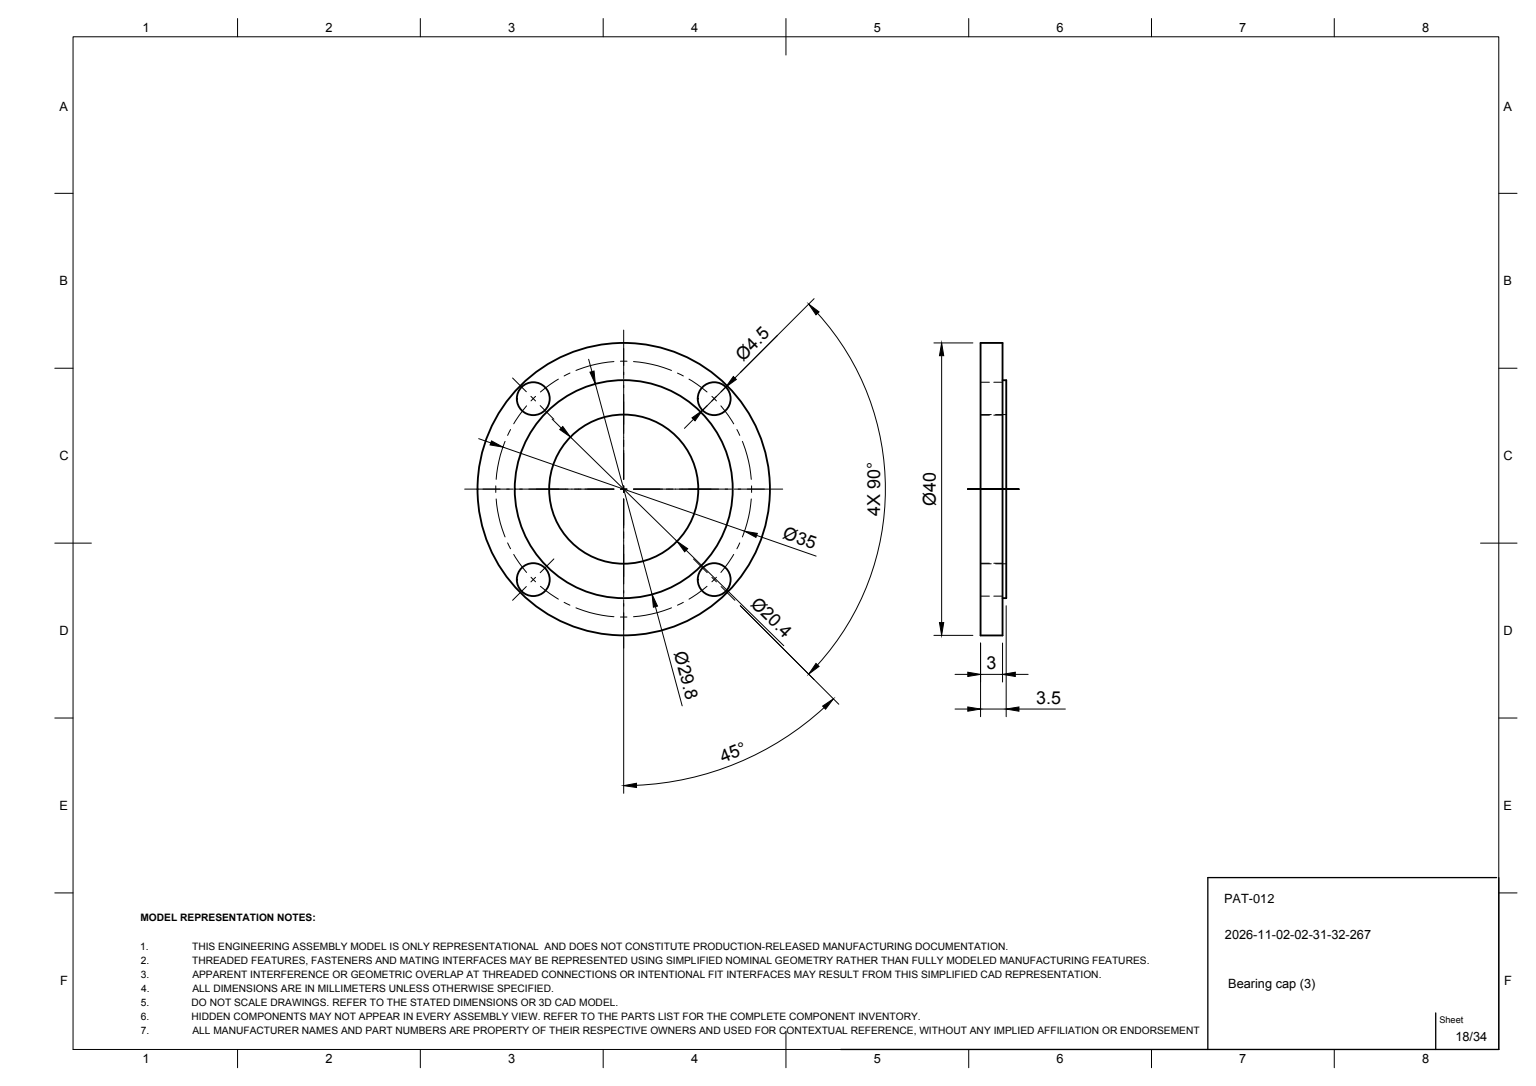
ISO-10303-21;
HEADER;
/* Generated by software containing ST-Developer
 * from STEP Tools, Inc. (www.steptools.com) 
 */

FILE_DESCRIPTION(
/* description */ ('Belt tensioner idler arm'),
/* implementation_level */ '2;1');

FILE_NAME(
/* name */ 'Bearing cap (3).step',
/* time_stamp */ '2026-10-28T03:22:15-07:00',
/* author */ (''),
/* organization */ (''),
/* preprocessor_version */ 'ST-DEVELOPER v20.2',
/* originating_system */ 'Autodesk Translation Framework v15.17.0.0',
/* authorisation */ '');

FILE_SCHEMA (('AUTOMOTIVE_DESIGN { 1 0 10303 214 3 1 1 }'));
ENDSEC;

DATA;
#10=MECHANICAL_DESIGN_GEOMETRIC_PRESENTATION_REPRESENTATION('',(#463),#12779);
#395=SHAPE_REPRESENTATION_RELATIONSHIP('SRR','None',#12942,#429);
#429=ADVANCED_BREP_SHAPE_REPRESENTATION('',(#503),#12759);
#463=STYLED_ITEM('',(#13184),#503);
#503=MANIFOLD_SOLID_BREP('Body1',#6199);
#615=FACE_BOUND('',#1463,.T.);
#616=FACE_BOUND('',#1467,.T.);
#617=FACE_BOUND('',#1468,.T.);
#618=FACE_BOUND('',#1469,.T.);
#619=FACE_BOUND('',#1470,.T.);
#620=FACE_BOUND('',#1471,.T.);
#621=FACE_BOUND('',#1473,.T.);
#622=FACE_BOUND('',#1474,.T.);
#623=FACE_BOUND('',#1475,.T.);
#624=FACE_BOUND('',#1476,.T.);
#625=FACE_BOUND('',#1477,.T.);
#753=PLANE('',#6941);
#754=PLANE('',#6948);
#755=PLANE('',#6949);
#1002=FACE_OUTER_BOUND('',#1457,.T.);
#1003=FACE_OUTER_BOUND('',#1458,.T.);
#1004=FACE_OUTER_BOUND('',#1459,.T.);
#1005=FACE_OUTER_BOUND('',#1460,.T.);
#1006=FACE_OUTER_BOUND('',#1461,.T.);
#1007=FACE_OUTER_BOUND('',#1462,.T.);
#1008=FACE_OUTER_BOUND('',#1464,.T.);
#1009=FACE_OUTER_BOUND('',#1465,.T.);
#1010=FACE_OUTER_BOUND('',#1466,.T.);
#1011=FACE_OUTER_BOUND('',#1472,.T.);
#1457=EDGE_LOOP('',(#4764,#4765,#4766,#4767));
#1458=EDGE_LOOP('',(#4768,#4769,#4770,#4771));
#1459=EDGE_LOOP('',(#4772,#4773,#4774,#4775));
#1460=EDGE_LOOP('',(#4776,#4777,#4778,#4779));
#1461=EDGE_LOOP('',(#4780,#4781,#4782,#4783));
#1462=EDGE_LOOP('',(#4784));
#1463=EDGE_LOOP('',(#4785));
#1464=EDGE_LOOP('',(#4786,#4787,#4788,#4789));
#1465=EDGE_LOOP('',(#4790,#4791,#4792,#4793));
#1466=EDGE_LOOP('',(#4794));
#1467=EDGE_LOOP('',(#4795));
#1468=EDGE_LOOP('',(#4796));
#1469=EDGE_LOOP('',(#4797));
#1470=EDGE_LOOP('',(#4798));
#1471=EDGE_LOOP('',(#4799));
#1472=EDGE_LOOP('',(#4800));
#1473=EDGE_LOOP('',(#4801));
#1474=EDGE_LOOP('',(#4802));
#1475=EDGE_LOOP('',(#4803));
#1476=EDGE_LOOP('',(#4804));
#1477=EDGE_LOOP('',(#4805));
#1882=LINE('',#10918,#2231);
#1883=LINE('',#10924,#2232);
#1884=LINE('',#10930,#2233);
#1885=LINE('',#10936,#2234);
#1886=LINE('',#10942,#2235);
#1887=LINE('',#10950,#2236);
#1888=LINE('',#10955,#2237);
#2231=VECTOR('',#8260,0.225);
#2232=VECTOR('',#8267,0.225);
#2233=VECTOR('',#8274,0.225);
#2234=VECTOR('',#8281,0.225);
#2235=VECTOR('',#8288,1.49);
#2236=VECTOR('',#8299,1.02);
#2237=VECTOR('',#8304,2.);
#2544=CIRCLE('',#6927,0.225);
#2545=CIRCLE('',#6928,0.225);
#2546=CIRCLE('',#6930,0.225);
#2547=CIRCLE('',#6931,0.225);
#2548=CIRCLE('',#6933,0.225);
#2549=CIRCLE('',#6934,0.225);
#2550=CIRCLE('',#6936,0.225);
#2551=CIRCLE('',#6937,0.225);
#2552=CIRCLE('',#6939,1.49);
#2553=CIRCLE('',#6940,1.49);
#2554=CIRCLE('',#6942,1.02);
#2555=CIRCLE('',#6944,1.02);
#2556=CIRCLE('',#6946,2.);
#2557=CIRCLE('',#6947,2.);
#2989=VERTEX_POINT('',#10915);
#2990=VERTEX_POINT('',#10917);
#2991=VERTEX_POINT('',#10921);
#2992=VERTEX_POINT('',#10923);
#2993=VERTEX_POINT('',#10927);
#2994=VERTEX_POINT('',#10929);
#2995=VERTEX_POINT('',#10933);
#2996=VERTEX_POINT('',#10935);
#2997=VERTEX_POINT('',#10939);
#2998=VERTEX_POINT('',#10941);
#2999=VERTEX_POINT('',#10945);
#3000=VERTEX_POINT('',#10948);
#3001=VERTEX_POINT('',#10952);
#3002=VERTEX_POINT('',#10954);
#3637=EDGE_CURVE('',#2989,#2989,#2544,.T.);
#3638=EDGE_CURVE('',#2989,#2990,#1882,.T.);
#3639=EDGE_CURVE('',#2990,#2990,#2545,.T.);
#3640=EDGE_CURVE('',#2991,#2991,#2546,.T.);
#3641=EDGE_CURVE('',#2991,#2992,#1883,.T.);
#3642=EDGE_CURVE('',#2992,#2992,#2547,.T.);
#3643=EDGE_CURVE('',#2993,#2993,#2548,.T.);
#3644=EDGE_CURVE('',#2993,#2994,#1884,.T.);
#3645=EDGE_CURVE('',#2994,#2994,#2549,.T.);
#3646=EDGE_CURVE('',#2995,#2995,#2550,.T.);
#3647=EDGE_CURVE('',#2995,#2996,#1885,.T.);
#3648=EDGE_CURVE('',#2996,#2996,#2551,.T.);
#3649=EDGE_CURVE('',#2997,#2997,#2552,.T.);
#3650=EDGE_CURVE('',#2997,#2998,#1886,.T.);
#3651=EDGE_CURVE('',#2998,#2998,#2553,.T.);
#3652=EDGE_CURVE('',#2999,#2999,#2554,.T.);
#3653=EDGE_CURVE('',#3000,#3000,#2555,.T.);
#3654=EDGE_CURVE('',#3000,#2999,#1887,.T.);
#3655=EDGE_CURVE('',#3001,#3001,#2556,.T.);
#3656=EDGE_CURVE('',#3001,#3002,#1888,.T.);
#3657=EDGE_CURVE('',#3002,#3002,#2557,.T.);
#4764=ORIENTED_EDGE('',*,*,#3637,.F.);
#4765=ORIENTED_EDGE('',*,*,#3638,.T.);
#4766=ORIENTED_EDGE('',*,*,#3639,.F.);
#4767=ORIENTED_EDGE('',*,*,#3638,.F.);
#4768=ORIENTED_EDGE('',*,*,#3640,.F.);
#4769=ORIENTED_EDGE('',*,*,#3641,.T.);
#4770=ORIENTED_EDGE('',*,*,#3642,.F.);
#4771=ORIENTED_EDGE('',*,*,#3641,.F.);
#4772=ORIENTED_EDGE('',*,*,#3643,.F.);
#4773=ORIENTED_EDGE('',*,*,#3644,.T.);
#4774=ORIENTED_EDGE('',*,*,#3645,.F.);
#4775=ORIENTED_EDGE('',*,*,#3644,.F.);
#4776=ORIENTED_EDGE('',*,*,#3646,.F.);
#4777=ORIENTED_EDGE('',*,*,#3647,.T.);
#4778=ORIENTED_EDGE('',*,*,#3648,.F.);
#4779=ORIENTED_EDGE('',*,*,#3647,.F.);
#4780=ORIENTED_EDGE('',*,*,#3649,.F.);
#4781=ORIENTED_EDGE('',*,*,#3650,.T.);
#4782=ORIENTED_EDGE('',*,*,#3651,.T.);
#4783=ORIENTED_EDGE('',*,*,#3650,.F.);
#4784=ORIENTED_EDGE('',*,*,#3651,.F.);
#4785=ORIENTED_EDGE('',*,*,#3652,.F.);
#4786=ORIENTED_EDGE('',*,*,#3653,.F.);
#4787=ORIENTED_EDGE('',*,*,#3654,.T.);
#4788=ORIENTED_EDGE('',*,*,#3652,.T.);
#4789=ORIENTED_EDGE('',*,*,#3654,.F.);
#4790=ORIENTED_EDGE('',*,*,#3655,.F.);
#4791=ORIENTED_EDGE('',*,*,#3656,.T.);
#4792=ORIENTED_EDGE('',*,*,#3657,.T.);
#4793=ORIENTED_EDGE('',*,*,#3656,.F.);
#4794=ORIENTED_EDGE('',*,*,#3655,.T.);
#4795=ORIENTED_EDGE('',*,*,#3653,.T.);
#4796=ORIENTED_EDGE('',*,*,#3648,.T.);
#4797=ORIENTED_EDGE('',*,*,#3645,.T.);
#4798=ORIENTED_EDGE('',*,*,#3642,.T.);
#4799=ORIENTED_EDGE('',*,*,#3639,.T.);
#4800=ORIENTED_EDGE('',*,*,#3657,.F.);
#4801=ORIENTED_EDGE('',*,*,#3649,.T.);
#4802=ORIENTED_EDGE('',*,*,#3646,.T.);
#4803=ORIENTED_EDGE('',*,*,#3643,.T.);
#4804=ORIENTED_EDGE('',*,*,#3640,.T.);
#4805=ORIENTED_EDGE('',*,*,#3637,.T.);
#5725=CYLINDRICAL_SURFACE('',#6926,0.225);
#5726=CYLINDRICAL_SURFACE('',#6929,0.225);
#5727=CYLINDRICAL_SURFACE('',#6932,0.225);
#5728=CYLINDRICAL_SURFACE('',#6935,0.225);
#5729=CYLINDRICAL_SURFACE('',#6938,1.49);
#5730=CYLINDRICAL_SURFACE('',#6943,1.02);
#5731=CYLINDRICAL_SURFACE('',#6945,2.);
#5979=ADVANCED_FACE('',(#1002),#5725,.F.);
#5980=ADVANCED_FACE('',(#1003),#5726,.F.);
#5981=ADVANCED_FACE('',(#1004),#5727,.F.);
#5982=ADVANCED_FACE('',(#1005),#5728,.F.);
#5983=ADVANCED_FACE('',(#1006),#5729,.T.);
#5984=ADVANCED_FACE('',(#1007,#615),#753,.F.);
#5985=ADVANCED_FACE('',(#1008),#5730,.F.);
#5986=ADVANCED_FACE('',(#1009),#5731,.T.);
#5987=ADVANCED_FACE('',(#1010,#616,#617,#618,#619,#620),#754,.T.);
#5988=ADVANCED_FACE('',(#1011,#621,#622,#623,#624,#625),#755,.F.);
#6199=CLOSED_SHELL('',(#5979,#5980,#5981,#5982,#5983,#5984,#5985,#5986,
#5987,#5988));
#6925=AXIS2_PLACEMENT_3D('',#10913,#8254,#8255);
#6926=AXIS2_PLACEMENT_3D('',#10914,#8256,#8257);
#6927=AXIS2_PLACEMENT_3D('',#10916,#8258,#8259);
#6928=AXIS2_PLACEMENT_3D('',#10919,#8261,#8262);
#6929=AXIS2_PLACEMENT_3D('',#10920,#8263,#8264);
#6930=AXIS2_PLACEMENT_3D('',#10922,#8265,#8266);
#6931=AXIS2_PLACEMENT_3D('',#10925,#8268,#8269);
#6932=AXIS2_PLACEMENT_3D('',#10926,#8270,#8271);
#6933=AXIS2_PLACEMENT_3D('',#10928,#8272,#8273);
#6934=AXIS2_PLACEMENT_3D('',#10931,#8275,#8276);
#6935=AXIS2_PLACEMENT_3D('',#10932,#8277,#8278);
#6936=AXIS2_PLACEMENT_3D('',#10934,#8279,#8280);
#6937=AXIS2_PLACEMENT_3D('',#10937,#8282,#8283);
#6938=AXIS2_PLACEMENT_3D('',#10938,#8284,#8285);
#6939=AXIS2_PLACEMENT_3D('',#10940,#8286,#8287);
#6940=AXIS2_PLACEMENT_3D('',#10943,#8289,#8290);
#6941=AXIS2_PLACEMENT_3D('',#10944,#8291,#8292);
#6942=AXIS2_PLACEMENT_3D('',#10946,#8293,#8294);
#6943=AXIS2_PLACEMENT_3D('',#10947,#8295,#8296);
#6944=AXIS2_PLACEMENT_3D('',#10949,#8297,#8298);
#6945=AXIS2_PLACEMENT_3D('',#10951,#8300,#8301);
#6946=AXIS2_PLACEMENT_3D('',#10953,#8302,#8303);
#6947=AXIS2_PLACEMENT_3D('',#10956,#8305,#8306);
#6948=AXIS2_PLACEMENT_3D('',#10957,#8307,#8308);
#6949=AXIS2_PLACEMENT_3D('',#10958,#8309,#8310);
#8254=DIRECTION('axis',(0.,0.,1.));
#8255=DIRECTION('refdir',(1.,0.,0.));
#8256=DIRECTION('center_axis',(0.,0.,1.));
#8257=DIRECTION('ref_axis',(1.,0.,0.));
#8258=DIRECTION('center_axis',(0.,0.,1.));
#8259=DIRECTION('ref_axis',(1.,0.,0.));
#8260=DIRECTION('',(0.,0.,1.));
#8261=DIRECTION('center_axis',(0.,0.,-1.));
#8262=DIRECTION('ref_axis',(1.,0.,0.));
#8263=DIRECTION('center_axis',(0.,0.,1.));
#8264=DIRECTION('ref_axis',(1.,0.,0.));
#8265=DIRECTION('center_axis',(0.,0.,1.));
#8266=DIRECTION('ref_axis',(1.,0.,0.));
#8267=DIRECTION('',(0.,0.,1.));
#8268=DIRECTION('center_axis',(0.,0.,-1.));
#8269=DIRECTION('ref_axis',(1.,0.,0.));
#8270=DIRECTION('center_axis',(0.,0.,1.));
#8271=DIRECTION('ref_axis',(1.,0.,0.));
#8272=DIRECTION('center_axis',(0.,0.,1.));
#8273=DIRECTION('ref_axis',(1.,0.,0.));
#8274=DIRECTION('',(0.,0.,1.));
#8275=DIRECTION('center_axis',(0.,0.,-1.));
#8276=DIRECTION('ref_axis',(1.,0.,0.));
#8277=DIRECTION('center_axis',(0.,0.,1.));
#8278=DIRECTION('ref_axis',(1.,0.,0.));
#8279=DIRECTION('center_axis',(0.,0.,1.));
#8280=DIRECTION('ref_axis',(1.,0.,0.));
#8281=DIRECTION('',(0.,0.,1.));
#8282=DIRECTION('center_axis',(0.,0.,-1.));
#8283=DIRECTION('ref_axis',(1.,0.,0.));
#8284=DIRECTION('center_axis',(0.,0.,1.));
#8285=DIRECTION('ref_axis',(1.,0.,0.));
#8286=DIRECTION('center_axis',(0.,0.,1.));
#8287=DIRECTION('ref_axis',(1.,0.,0.));
#8288=DIRECTION('',(0.,0.,-1.));
#8289=DIRECTION('center_axis',(0.,0.,1.));
#8290=DIRECTION('ref_axis',(1.,0.,0.));
#8291=DIRECTION('center_axis',(0.,0.,1.));
#8292=DIRECTION('ref_axis',(1.,0.,0.));
#8293=DIRECTION('center_axis',(0.,0.,-1.));
#8294=DIRECTION('ref_axis',(1.,0.,0.));
#8295=DIRECTION('center_axis',(0.,0.,1.));
#8296=DIRECTION('ref_axis',(1.,0.,0.));
#8297=DIRECTION('center_axis',(0.,0.,-1.));
#8298=DIRECTION('ref_axis',(1.,0.,0.));
#8299=DIRECTION('',(0.,0.,-1.));
#8300=DIRECTION('center_axis',(0.,0.,1.));
#8301=DIRECTION('ref_axis',(1.,0.,0.));
#8302=DIRECTION('center_axis',(0.,0.,1.));
#8303=DIRECTION('ref_axis',(1.,0.,0.));
#8304=DIRECTION('',(0.,0.,-1.));
#8305=DIRECTION('center_axis',(0.,0.,1.));
#8306=DIRECTION('ref_axis',(1.,0.,0.));
#8307=DIRECTION('center_axis',(0.,0.,1.));
#8308=DIRECTION('ref_axis',(1.,0.,0.));
#8309=DIRECTION('center_axis',(0.,0.,1.));
#8310=DIRECTION('ref_axis',(1.,0.,0.));
#10913=CARTESIAN_POINT('',(0.,0.,0.));
#10914=CARTESIAN_POINT('Origin',(7.76256313292354,-1.23743686707646,5.9));
#10915=CARTESIAN_POINT('',(7.53756313292354,-1.23743686707646,6.));
#10916=CARTESIAN_POINT('Origin',(7.76256313292354,-1.23743686707646,6.));
#10917=CARTESIAN_POINT('',(7.53756313292354,-1.23743686707646,6.3));
#10918=CARTESIAN_POINT('',(7.53756313292354,-1.23743686707646,5.9));
#10919=CARTESIAN_POINT('Origin',(7.76256313292354,-1.23743686707646,6.3));
#10920=CARTESIAN_POINT('Origin',(7.76256313292354,1.23743686707646,5.9));
#10921=CARTESIAN_POINT('',(7.53756313292354,1.23743686707646,6.));
#10922=CARTESIAN_POINT('Origin',(7.76256313292354,1.23743686707646,6.));
#10923=CARTESIAN_POINT('',(7.53756313292354,1.23743686707646,6.3));
#10924=CARTESIAN_POINT('',(7.53756313292354,1.23743686707646,5.9));
#10925=CARTESIAN_POINT('Origin',(7.76256313292354,1.23743686707646,6.3));
#10926=CARTESIAN_POINT('Origin',(10.2374368670765,1.23743686707646,5.9));
#10927=CARTESIAN_POINT('',(10.0124368670765,1.23743686707646,6.));
#10928=CARTESIAN_POINT('Origin',(10.2374368670765,1.23743686707646,6.));
#10929=CARTESIAN_POINT('',(10.0124368670765,1.23743686707646,6.3));
#10930=CARTESIAN_POINT('',(10.0124368670765,1.23743686707646,5.9));
#10931=CARTESIAN_POINT('Origin',(10.2374368670765,1.23743686707646,6.3));
#10932=CARTESIAN_POINT('Origin',(10.2374368670765,-1.23743686707646,5.9));
#10933=CARTESIAN_POINT('',(10.0124368670765,-1.23743686707646,6.));
#10934=CARTESIAN_POINT('Origin',(10.2374368670765,-1.23743686707646,6.));
#10935=CARTESIAN_POINT('',(10.0124368670765,-1.23743686707646,6.3));
#10936=CARTESIAN_POINT('',(10.0124368670765,-1.23743686707646,5.9));
#10937=CARTESIAN_POINT('Origin',(10.2374368670765,-1.23743686707646,6.3));
#10938=CARTESIAN_POINT('Origin',(9.,0.,5.95));
#10939=CARTESIAN_POINT('',(7.51,-1.82472373072956E-16,6.));
#10940=CARTESIAN_POINT('Origin',(9.,0.,6.));
#10941=CARTESIAN_POINT('',(7.51,-1.82472373072956E-16,5.95));
#10942=CARTESIAN_POINT('',(7.51,-1.82472373072956E-16,5.95));
#10943=CARTESIAN_POINT('Origin',(9.,0.,5.95));
#10944=CARTESIAN_POINT('Origin',(9.,0.,5.95));
#10945=CARTESIAN_POINT('',(7.98,-1.2491397351303E-16,5.95));
#10946=CARTESIAN_POINT('Origin',(9.,0.,5.95));
#10947=CARTESIAN_POINT('Origin',(9.,0.,6.));
#10948=CARTESIAN_POINT('',(7.98,-1.2491397351303E-16,6.3));
#10949=CARTESIAN_POINT('Origin',(9.,0.,6.3));
#10950=CARTESIAN_POINT('',(7.98,-1.2491397351303E-16,6.));
#10951=CARTESIAN_POINT('Origin',(9.,0.,6.));
#10952=CARTESIAN_POINT('',(7.,-2.44929359829471E-16,6.3));
#10953=CARTESIAN_POINT('Origin',(9.,0.,6.3));
#10954=CARTESIAN_POINT('',(7.,-2.44929359829471E-16,6.));
#10955=CARTESIAN_POINT('',(7.,-2.44929359829471E-16,6.));
#10956=CARTESIAN_POINT('Origin',(9.,0.,6.));
#10957=CARTESIAN_POINT('Origin',(9.,0.,6.3));
#10958=CARTESIAN_POINT('Origin',(9.,0.,6.));
#12719=UNCERTAINTY_MEASURE_WITH_UNIT(LENGTH_MEASURE(0.001),#12780,
'DISTANCE_ACCURACY_VALUE',
'Maximum model space distance between geometric entities at asserted c
onnectivities');
#12739=UNCERTAINTY_MEASURE_WITH_UNIT(LENGTH_MEASURE(0.001),#12780,
'DISTANCE_ACCURACY_VALUE',
'Maximum model space distance between geometric entities at asserted c
onnectivities');
#12759=(
GEOMETRIC_REPRESENTATION_CONTEXT(3)
GLOBAL_UNCERTAINTY_ASSIGNED_CONTEXT((#12719))
GLOBAL_UNIT_ASSIGNED_CONTEXT((#12780,#12782,#12783))
REPRESENTATION_CONTEXT('','3D')
);
#12779=(
GEOMETRIC_REPRESENTATION_CONTEXT(3)
GLOBAL_UNCERTAINTY_ASSIGNED_CONTEXT((#12739))
GLOBAL_UNIT_ASSIGNED_CONTEXT((#12780,#12782,#12783))
REPRESENTATION_CONTEXT('','3D')
);
#12780=(
LENGTH_UNIT()
NAMED_UNIT(*)
SI_UNIT(.CENTI.,.METRE.)
);
#12782=(
NAMED_UNIT(*)
PLANE_ANGLE_UNIT()
SI_UNIT($,.RADIAN.)
);
#12783=(
NAMED_UNIT(*)
SI_UNIT($,.STERADIAN.)
SOLID_ANGLE_UNIT()
);
#12803=SHAPE_DEFINITION_REPRESENTATION(#12842,#12942);
#12842=PRODUCT_DEFINITION_SHAPE('',$,#12982);
#12942=SHAPE_REPRESENTATION('',(#6925),#12759);
#12962=PRODUCT_DEFINITION_CONTEXT('part definition',#13081,'design');
#12982=PRODUCT_DEFINITION('Bearing cap (3)','Bearing cap (3)',#13021,#12962);
#13021=PRODUCT_DEFINITION_FORMATION('',$,#13102);
#13081=APPLICATION_CONTEXT(
'Core Data for Automotive Mechanical Design Process');
#13082=PRODUCT_CONTEXT('part definition',#13081,'mechanical');
#13102=PRODUCT('Bearing cap (3)','Bearing cap (3)','Bearing cap (3)',(#13082));
#13178=COLOUR_RGB('Grey',0.48,0.52,0.57);
#13179=FILL_AREA_STYLE_COLOUR('',#13178);
#13180=FILL_AREA_STYLE('',(#13179));
#13181=SURFACE_STYLE_FILL_AREA(#13180);
#13182=SURFACE_SIDE_STYLE('',(#13181));
#13183=SURFACE_STYLE_USAGE(.BOTH.,#13182);
#13184=PRESENTATION_STYLE_ASSIGNMENT((#13183));
ENDSEC;
END-ISO-10303-21;
